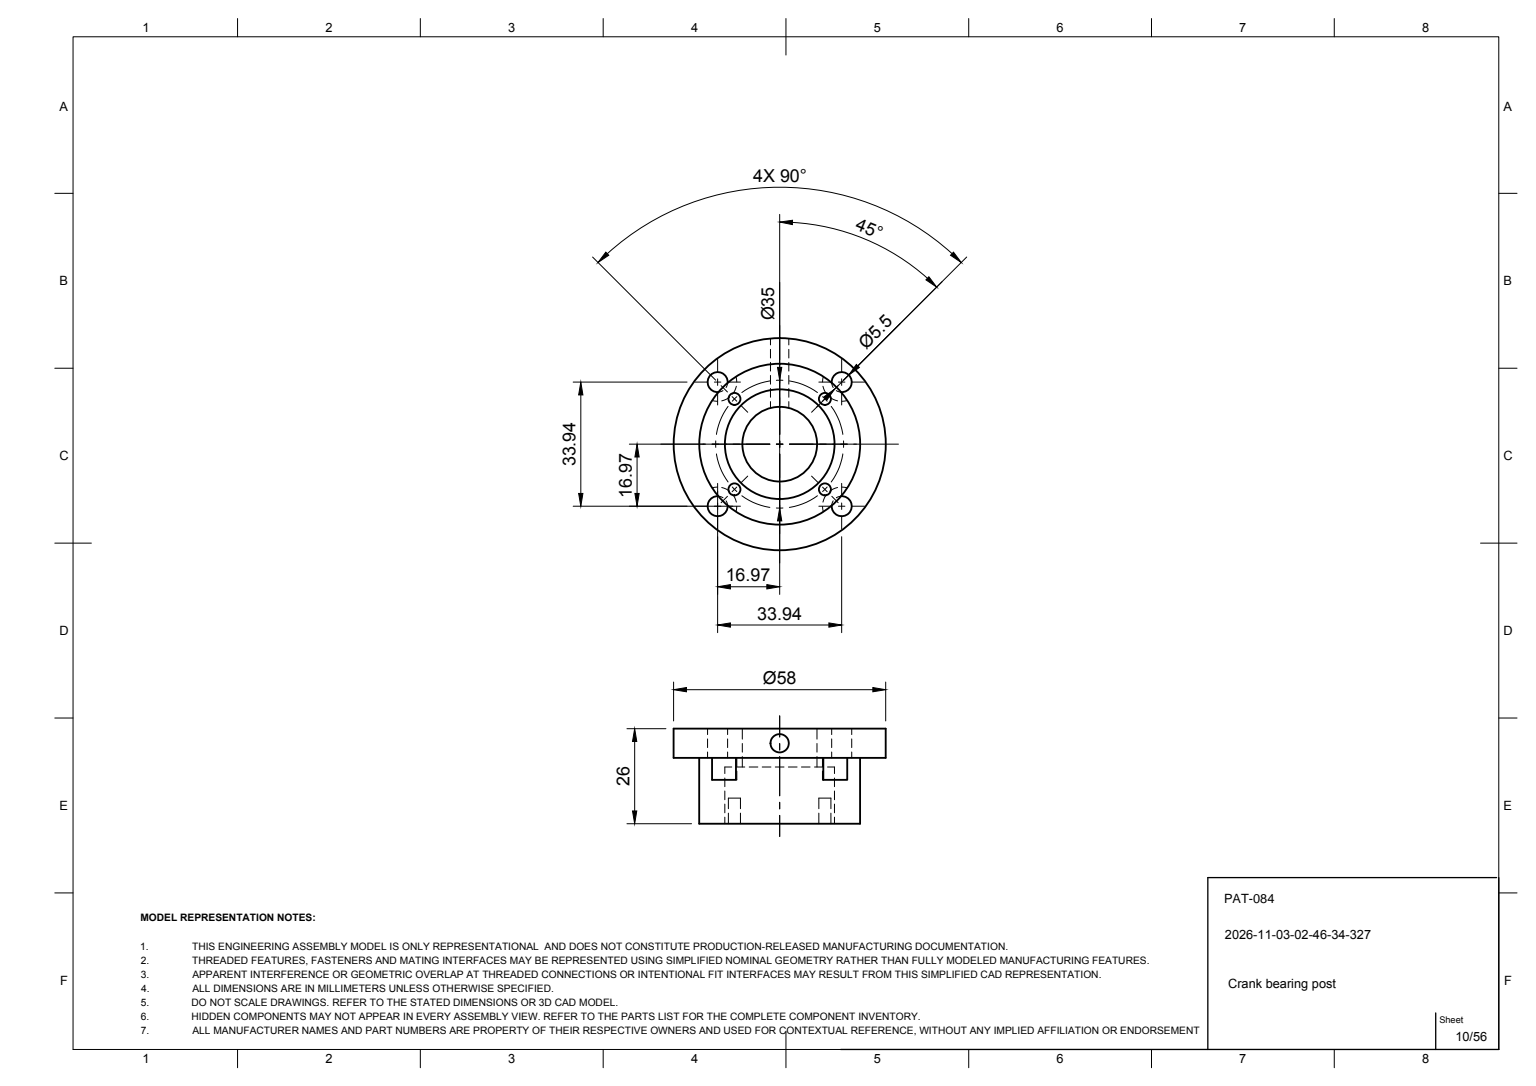
ISO-10303-21;
HEADER;
/* Generated by software containing ST-Developer
 * from STEP Tools, Inc. (www.steptools.com) 
 */

FILE_DESCRIPTION(
/* description */ ('Quick-return (Whitworth) mechanism'),
/* implementation_level */ '2;1');

FILE_NAME(
/* name */ 'Crank bearing post.step',
/* time_stamp */ '2026-10-28T03:25:57-07:00',
/* author */ (''),
/* organization */ (''),
/* preprocessor_version */ 'ST-DEVELOPER v20.2',
/* originating_system */ 'Autodesk Translation Framework v15.17.0.0',
/* authorisation */ '');

FILE_SCHEMA (('AUTOMOTIVE_DESIGN { 1 0 10303 214 3 1 1 }'));
ENDSEC;

DATA;
#10=MECHANICAL_DESIGN_GEOMETRIC_PRESENTATION_REPRESENTATION('',(#495),#14878);
#370=B_SPLINE_CURVE_WITH_KNOTS('',3,(#12386,#12387,#12388,#12389,#12390,
#12391,#12392,#12393,#12394,#12395),.UNSPECIFIED.,.F.,.F.,(4,2,2,2,4),(0.,
0.094594182476448,0.189188364952896,0.283770357603024,0.378352350253152),
 .UNSPECIFIED.);
#371=B_SPLINE_CURVE_WITH_KNOTS('',3,(#12396,#12397,#12398,#12399,#12400,
#12401,#12402,#12403,#12404,#12405,#12406,#12407,#12408,#12409,#12410,#12411,
#12412,#12413,#12414,#12415,#12416,#12417,#12418,#12419,#12420,#12421),
 .UNSPECIFIED.,.F.,.F.,(4,2,2,2,2,2,2,2,2,2,2,2,4),(0.378352350253152,0.472934342903279,
0.567516335553407,0.662110518029855,0.756704700506303,0.851298882982751,
0.945893065459199,1.04047505810933,1.13505705075945,1.22963904340958,1.32422103605971,
1.41881521853616,1.51340940101261),.UNSPECIFIED.);
#372=B_SPLINE_CURVE_WITH_KNOTS('',3,(#12425,#12426,#12427,#12428,#12429,
#12430,#12431,#12432,#12433,#12434,#12435,#12436,#12437,#12438,#12439,#12440,
#12441,#12442,#12443,#12444,#12445,#12446,#12447,#12448,#12449,#12450),
 .UNSPECIFIED.,.F.,.F.,(4,2,2,2,2,2,2,2,2,2,2,2,4),(0.,0.094221953570005,
0.18844390714001,0.282665684012033,0.376887460884057,0.47110923775608,0.565331014628104,
0.659552968198109,0.753774921768114,0.847996875338119,0.942218828908123,
1.03644060578015,1.13066238265217),.UNSPECIFIED.);
#373=B_SPLINE_CURVE_WITH_KNOTS('',3,(#12451,#12452,#12453,#12454,#12455,
#12456,#12457,#12458,#12459,#12460),.UNSPECIFIED.,.F.,.F.,(4,2,2,2,4),(1.13066238265217,
1.22488415952419,1.31910593639622,1.41332788996622,1.50754984353623),
 .UNSPECIFIED.);
#407=SHAPE_REPRESENTATION_RELATIONSHIP('SRR','None',#15075,#451);
#451=ADVANCED_BREP_SHAPE_REPRESENTATION('',(#547),#14832);
#495=STYLED_ITEM('',(#15406),#547);
#547=MANIFOLD_SOLID_BREP('Body1',#7849);
#648=FACE_BOUND('',#1665,.T.);
#649=FACE_BOUND('',#1666,.T.);
#650=FACE_BOUND('',#1667,.T.);
#651=FACE_BOUND('',#1668,.T.);
#652=FACE_BOUND('',#1669,.T.);
#653=FACE_BOUND('',#1677,.T.);
#654=FACE_BOUND('',#1679,.T.);
#655=FACE_BOUND('',#1681,.T.);
#656=FACE_BOUND('',#1683,.T.);
#657=FACE_BOUND('',#1684,.T.);
#658=FACE_BOUND('',#1685,.T.);
#659=FACE_BOUND('',#1686,.T.);
#660=FACE_BOUND('',#1687,.T.);
#661=FACE_BOUND('',#1689,.T.);
#662=FACE_BOUND('',#1690,.T.);
#663=FACE_BOUND('',#1691,.T.);
#664=FACE_BOUND('',#1692,.T.);
#665=FACE_BOUND('',#1693,.T.);
#819=PLANE('',#8559);
#820=PLANE('',#8563);
#821=PLANE('',#8567);
#822=PLANE('',#8571);
#823=PLANE('',#8575);
#824=PLANE('',#8580);
#825=PLANE('',#8585);
#826=PLANE('',#8590);
#827=PLANE('',#8592);
#828=PLANE('',#8616);
#829=PLANE('',#8622);
#830=PLANE('',#8623);
#1124=FACE_OUTER_BOUND('',#1647,.T.);
#1125=FACE_OUTER_BOUND('',#1648,.T.);
#1126=FACE_OUTER_BOUND('',#1649,.T.);
#1127=FACE_OUTER_BOUND('',#1650,.T.);
#1128=FACE_OUTER_BOUND('',#1651,.T.);
#1129=FACE_OUTER_BOUND('',#1652,.T.);
#1130=FACE_OUTER_BOUND('',#1653,.T.);
#1131=FACE_OUTER_BOUND('',#1654,.T.);
#1132=FACE_OUTER_BOUND('',#1655,.T.);
#1133=FACE_OUTER_BOUND('',#1656,.T.);
#1134=FACE_OUTER_BOUND('',#1657,.T.);
#1135=FACE_OUTER_BOUND('',#1658,.T.);
#1136=FACE_OUTER_BOUND('',#1659,.T.);
#1137=FACE_OUTER_BOUND('',#1660,.T.);
#1138=FACE_OUTER_BOUND('',#1661,.T.);
#1139=FACE_OUTER_BOUND('',#1662,.T.);
#1140=FACE_OUTER_BOUND('',#1663,.T.);
#1141=FACE_OUTER_BOUND('',#1664,.T.);
#1142=FACE_OUTER_BOUND('',#1670,.T.);
#1143=FACE_OUTER_BOUND('',#1671,.T.);
#1144=FACE_OUTER_BOUND('',#1672,.T.);
#1145=FACE_OUTER_BOUND('',#1673,.T.);
#1146=FACE_OUTER_BOUND('',#1674,.T.);
#1147=FACE_OUTER_BOUND('',#1675,.T.);
#1148=FACE_OUTER_BOUND('',#1676,.T.);
#1149=FACE_OUTER_BOUND('',#1678,.T.);
#1150=FACE_OUTER_BOUND('',#1680,.T.);
#1151=FACE_OUTER_BOUND('',#1682,.T.);
#1152=FACE_OUTER_BOUND('',#1688,.T.);
#1647=EDGE_LOOP('',(#5602,#5603,#5604,#5605,#5606,#5607));
#1648=EDGE_LOOP('',(#5608,#5609,#5610,#5611));
#1649=EDGE_LOOP('',(#5612));
#1650=EDGE_LOOP('',(#5613,#5614,#5615,#5616));
#1651=EDGE_LOOP('',(#5617));
#1652=EDGE_LOOP('',(#5618,#5619,#5620,#5621));
#1653=EDGE_LOOP('',(#5622));
#1654=EDGE_LOOP('',(#5623,#5624,#5625,#5626));
#1655=EDGE_LOOP('',(#5627));
#1656=EDGE_LOOP('',(#5628,#5629,#5630,#5631));
#1657=EDGE_LOOP('',(#5632,#5633));
#1658=EDGE_LOOP('',(#5634,#5635,#5636,#5637));
#1659=EDGE_LOOP('',(#5638,#5639));
#1660=EDGE_LOOP('',(#5640,#5641,#5642,#5643));
#1661=EDGE_LOOP('',(#5644,#5645));
#1662=EDGE_LOOP('',(#5646,#5647,#5648,#5649));
#1663=EDGE_LOOP('',(#5650,#5651));
#1664=EDGE_LOOP('',(#5652));
#1665=EDGE_LOOP('',(#5653,#5654,#5655,#5656,#5657,#5658,#5659,#5660,#5661));
#1666=EDGE_LOOP('',(#5662));
#1667=EDGE_LOOP('',(#5663));
#1668=EDGE_LOOP('',(#5664));
#1669=EDGE_LOOP('',(#5665));
#1670=EDGE_LOOP('',(#5666,#5667,#5668,#5669));
#1671=EDGE_LOOP('',(#5670,#5671,#5672,#5673));
#1672=EDGE_LOOP('',(#5674,#5675,#5676,#5677));
#1673=EDGE_LOOP('',(#5678,#5679,#5680,#5681));
#1674=EDGE_LOOP('',(#5682,#5683,#5684,#5685,#5686,#5687,#5688,#5689,#5690,
#5691,#5692,#5693,#5694,#5695,#5696,#5697,#5698,#5699,#5700,#5701));
#1675=EDGE_LOOP('',(#5702,#5703,#5704,#5705));
#1676=EDGE_LOOP('',(#5706));
#1677=EDGE_LOOP('',(#5707));
#1678=EDGE_LOOP('',(#5708,#5709,#5710,#5711));
#1679=EDGE_LOOP('',(#5712,#5713));
#1680=EDGE_LOOP('',(#5714,#5715,#5716,#5717));
#1681=EDGE_LOOP('',(#5718,#5719));
#1682=EDGE_LOOP('',(#5720));
#1683=EDGE_LOOP('',(#5721));
#1684=EDGE_LOOP('',(#5722));
#1685=EDGE_LOOP('',(#5723));
#1686=EDGE_LOOP('',(#5724));
#1687=EDGE_LOOP('',(#5725));
#1688=EDGE_LOOP('',(#5726));
#1689=EDGE_LOOP('',(#5727));
#1690=EDGE_LOOP('',(#5728));
#1691=EDGE_LOOP('',(#5729));
#1692=EDGE_LOOP('',(#5730));
#1693=EDGE_LOOP('',(#5731));
#2250=LINE('',#12423,#2773);
#2251=LINE('',#12465,#2774);
#2252=LINE('',#12472,#2775);
#2253=LINE('',#12479,#2776);
#2254=LINE('',#12486,#2777);
#2255=LINE('',#12492,#2778);
#2256=LINE('',#12496,#2779);
#2257=LINE('',#12503,#2780);
#2258=LINE('',#12507,#2781);
#2259=LINE('',#12514,#2782);
#2260=LINE('',#12518,#2783);
#2261=LINE('',#12525,#2784);
#2262=LINE('',#12529,#2785);
#2263=LINE('',#12553,#2786);
#2264=LINE('',#12557,#2787);
#2265=LINE('',#12561,#2788);
#2266=LINE('',#12565,#2789);
#2267=LINE('',#12569,#2790);
#2268=LINE('',#12574,#2791);
#2269=LINE('',#12581,#2792);
#2270=LINE('',#12585,#2793);
#2773=VECTOR('',#9821,0.25);
#2774=VECTOR('',#9826,0.165);
#2775=VECTOR('',#9835,0.165);
#2776=VECTOR('',#9844,0.165);
#2777=VECTOR('',#9853,0.165);
#2778=VECTOR('',#9860,1.);
#2779=VECTOR('',#9863,1.);
#2780=VECTOR('',#9872,1.);
#2781=VECTOR('',#9875,1.);
#2782=VECTOR('',#9884,1.);
#2783=VECTOR('',#9887,1.);
#2784=VECTOR('',#9896,1.);
#2785=VECTOR('',#9899,1.);
#2786=VECTOR('',#9932,0.275);
#2787=VECTOR('',#9937,0.275);
#2788=VECTOR('',#9942,0.275);
#2789=VECTOR('',#9947,0.275);
#2790=VECTOR('',#9952,2.2);
#2791=VECTOR('',#9957,1.5);
#2792=VECTOR('',#9966,2.9);
#2793=VECTOR('',#9971,1.02);
#3302=CIRCLE('',#8557,0.165);
#3303=CIRCLE('',#8558,0.165);
#3304=CIRCLE('',#8561,0.165);
#3305=CIRCLE('',#8562,0.165);
#3306=CIRCLE('',#8565,0.165);
#3307=CIRCLE('',#8566,0.165);
#3308=CIRCLE('',#8569,0.165);
#3309=CIRCLE('',#8570,0.165);
#3310=CIRCLE('',#8573,0.525);
#3311=CIRCLE('',#8574,0.525);
#3312=CIRCLE('',#8576,2.2);
#3313=CIRCLE('',#8578,0.525);
#3314=CIRCLE('',#8579,0.525);
#3315=CIRCLE('',#8581,2.2);
#3316=CIRCLE('',#8583,0.525);
#3317=CIRCLE('',#8584,0.525);
#3318=CIRCLE('',#8586,2.2);
#3319=CIRCLE('',#8588,0.525);
#3320=CIRCLE('',#8589,0.525);
#3321=CIRCLE('',#8591,2.2);
#3322=CIRCLE('',#8593,2.9);
#3323=CIRCLE('',#8594,2.2);
#3324=CIRCLE('',#8595,2.2);
#3325=CIRCLE('',#8596,2.2);
#3326=CIRCLE('',#8597,2.2);
#3327=CIRCLE('',#8598,2.2);
#3328=CIRCLE('',#8599,0.275);
#3329=CIRCLE('',#8600,0.275);
#3330=CIRCLE('',#8601,0.275);
#3331=CIRCLE('',#8602,0.275);
#3332=CIRCLE('',#8604,0.275);
#3333=CIRCLE('',#8606,0.275);
#3334=CIRCLE('',#8608,0.275);
#3335=CIRCLE('',#8610,0.275);
#3336=CIRCLE('',#8612,2.2);
#3337=CIRCLE('',#8614,1.5);
#3338=CIRCLE('',#8615,1.5);
#3339=CIRCLE('',#8617,1.02);
#3340=CIRCLE('',#8619,2.9);
#3341=CIRCLE('',#8621,1.02);
#3745=VERTEX_POINT('',#12384);
#3746=VERTEX_POINT('',#12385);
#3747=VERTEX_POINT('',#12422);
#3748=VERTEX_POINT('',#12424);
#3749=VERTEX_POINT('',#12462);
#3750=VERTEX_POINT('',#12464);
#3751=VERTEX_POINT('',#12469);
#3752=VERTEX_POINT('',#12471);
#3753=VERTEX_POINT('',#12476);
#3754=VERTEX_POINT('',#12478);
#3755=VERTEX_POINT('',#12483);
#3756=VERTEX_POINT('',#12485);
#3757=VERTEX_POINT('',#12490);
#3758=VERTEX_POINT('',#12491);
#3759=VERTEX_POINT('',#12493);
#3760=VERTEX_POINT('',#12495);
#3761=VERTEX_POINT('',#12501);
#3762=VERTEX_POINT('',#12502);
#3763=VERTEX_POINT('',#12504);
#3764=VERTEX_POINT('',#12506);
#3765=VERTEX_POINT('',#12512);
#3766=VERTEX_POINT('',#12513);
#3767=VERTEX_POINT('',#12515);
#3768=VERTEX_POINT('',#12517);
#3769=VERTEX_POINT('',#12523);
#3770=VERTEX_POINT('',#12524);
#3771=VERTEX_POINT('',#12526);
#3772=VERTEX_POINT('',#12528);
#3773=VERTEX_POINT('',#12534);
#3774=VERTEX_POINT('',#12536);
#3775=VERTEX_POINT('',#12542);
#3776=VERTEX_POINT('',#12544);
#3777=VERTEX_POINT('',#12546);
#3778=VERTEX_POINT('',#12548);
#3779=VERTEX_POINT('',#12551);
#3780=VERTEX_POINT('',#12555);
#3781=VERTEX_POINT('',#12559);
#3782=VERTEX_POINT('',#12563);
#3783=VERTEX_POINT('',#12567);
#3784=VERTEX_POINT('',#12571);
#3785=VERTEX_POINT('',#12573);
#3786=VERTEX_POINT('',#12577);
#3787=VERTEX_POINT('',#12580);
#3788=VERTEX_POINT('',#12584);
#4458=EDGE_CURVE('',#3745,#3746,#370,.T.);
#4459=EDGE_CURVE('',#3746,#3745,#371,.T.);
#4460=EDGE_CURVE('',#3746,#3747,#2250,.T.);
#4461=EDGE_CURVE('',#3748,#3747,#372,.T.);
#4462=EDGE_CURVE('',#3747,#3748,#373,.T.);
#4463=EDGE_CURVE('',#3749,#3749,#3302,.T.);
#4464=EDGE_CURVE('',#3749,#3750,#2251,.T.);
#4465=EDGE_CURVE('',#3750,#3750,#3303,.T.);
#4466=EDGE_CURVE('',#3751,#3751,#3304,.T.);
#4467=EDGE_CURVE('',#3751,#3752,#2252,.T.);
#4468=EDGE_CURVE('',#3752,#3752,#3305,.T.);
#4469=EDGE_CURVE('',#3753,#3753,#3306,.T.);
#4470=EDGE_CURVE('',#3753,#3754,#2253,.T.);
#4471=EDGE_CURVE('',#3754,#3754,#3307,.T.);
#4472=EDGE_CURVE('',#3755,#3755,#3308,.T.);
#4473=EDGE_CURVE('',#3755,#3756,#2254,.T.);
#4474=EDGE_CURVE('',#3756,#3756,#3309,.T.);
#4475=EDGE_CURVE('',#3757,#3758,#2255,.T.);
#4476=EDGE_CURVE('',#3757,#3759,#3310,.T.);
#4477=EDGE_CURVE('',#3760,#3759,#2256,.T.);
#4478=EDGE_CURVE('',#3758,#3760,#3311,.T.);
#4479=EDGE_CURVE('',#3759,#3757,#3312,.T.);
#4480=EDGE_CURVE('',#3761,#3762,#2257,.T.);
#4481=EDGE_CURVE('',#3761,#3763,#3313,.T.);
#4482=EDGE_CURVE('',#3764,#3763,#2258,.T.);
#4483=EDGE_CURVE('',#3762,#3764,#3314,.T.);
#4484=EDGE_CURVE('',#3763,#3761,#3315,.T.);
#4485=EDGE_CURVE('',#3765,#3766,#2259,.T.);
#4486=EDGE_CURVE('',#3765,#3767,#3316,.T.);
#4487=EDGE_CURVE('',#3768,#3767,#2260,.T.);
#4488=EDGE_CURVE('',#3766,#3768,#3317,.T.);
#4489=EDGE_CURVE('',#3767,#3765,#3318,.T.);
#4490=EDGE_CURVE('',#3769,#3770,#2261,.T.);
#4491=EDGE_CURVE('',#3769,#3771,#3319,.T.);
#4492=EDGE_CURVE('',#3772,#3771,#2262,.T.);
#4493=EDGE_CURVE('',#3770,#3772,#3320,.T.);
#4494=EDGE_CURVE('',#3771,#3769,#3321,.T.);
#4495=EDGE_CURVE('',#3773,#3773,#3322,.T.);
#4496=EDGE_CURVE('',#3762,#3774,#3323,.T.);
#4497=EDGE_CURVE('',#3766,#3764,#3324,.T.);
#4498=EDGE_CURVE('',#3770,#3768,#3325,.T.);
#4499=EDGE_CURVE('',#3758,#3772,#3326,.T.);
#4500=EDGE_CURVE('',#3774,#3760,#3327,.T.);
#4501=EDGE_CURVE('',#3775,#3775,#3328,.T.);
#4502=EDGE_CURVE('',#3776,#3776,#3329,.T.);
#4503=EDGE_CURVE('',#3777,#3777,#3330,.T.);
#4504=EDGE_CURVE('',#3778,#3778,#3331,.T.);
#4505=EDGE_CURVE('',#3779,#3779,#3332,.T.);
#4506=EDGE_CURVE('',#3779,#3775,#2263,.T.);
#4507=EDGE_CURVE('',#3780,#3780,#3333,.T.);
#4508=EDGE_CURVE('',#3780,#3776,#2264,.T.);
#4509=EDGE_CURVE('',#3781,#3781,#3334,.T.);
#4510=EDGE_CURVE('',#3781,#3777,#2265,.T.);
#4511=EDGE_CURVE('',#3782,#3782,#3335,.T.);
#4512=EDGE_CURVE('',#3782,#3778,#2266,.T.);
#4513=EDGE_CURVE('',#3783,#3783,#3336,.T.);
#4514=EDGE_CURVE('',#3783,#3774,#2267,.T.);
#4515=EDGE_CURVE('',#3784,#3784,#3337,.T.);
#4516=EDGE_CURVE('',#3784,#3785,#2268,.T.);
#4517=EDGE_CURVE('',#3785,#3785,#3338,.T.);
#4518=EDGE_CURVE('',#3786,#3786,#3339,.T.);
#4519=EDGE_CURVE('',#3773,#3787,#2269,.T.);
#4520=EDGE_CURVE('',#3787,#3787,#3340,.T.);
#4521=EDGE_CURVE('',#3786,#3788,#2270,.T.);
#4522=EDGE_CURVE('',#3788,#3788,#3341,.T.);
#5602=ORIENTED_EDGE('',*,*,#4458,.F.);
#5603=ORIENTED_EDGE('',*,*,#4459,.F.);
#5604=ORIENTED_EDGE('',*,*,#4460,.T.);
#5605=ORIENTED_EDGE('',*,*,#4461,.F.);
#5606=ORIENTED_EDGE('',*,*,#4462,.F.);
#5607=ORIENTED_EDGE('',*,*,#4460,.F.);
#5608=ORIENTED_EDGE('',*,*,#4463,.F.);
#5609=ORIENTED_EDGE('',*,*,#4464,.T.);
#5610=ORIENTED_EDGE('',*,*,#4465,.F.);
#5611=ORIENTED_EDGE('',*,*,#4464,.F.);
#5612=ORIENTED_EDGE('',*,*,#4463,.T.);
#5613=ORIENTED_EDGE('',*,*,#4466,.F.);
#5614=ORIENTED_EDGE('',*,*,#4467,.T.);
#5615=ORIENTED_EDGE('',*,*,#4468,.F.);
#5616=ORIENTED_EDGE('',*,*,#4467,.F.);
#5617=ORIENTED_EDGE('',*,*,#4466,.T.);
#5618=ORIENTED_EDGE('',*,*,#4469,.F.);
#5619=ORIENTED_EDGE('',*,*,#4470,.T.);
#5620=ORIENTED_EDGE('',*,*,#4471,.F.);
#5621=ORIENTED_EDGE('',*,*,#4470,.F.);
#5622=ORIENTED_EDGE('',*,*,#4469,.T.);
#5623=ORIENTED_EDGE('',*,*,#4472,.F.);
#5624=ORIENTED_EDGE('',*,*,#4473,.T.);
#5625=ORIENTED_EDGE('',*,*,#4474,.F.);
#5626=ORIENTED_EDGE('',*,*,#4473,.F.);
#5627=ORIENTED_EDGE('',*,*,#4472,.T.);
#5628=ORIENTED_EDGE('',*,*,#4475,.F.);
#5629=ORIENTED_EDGE('',*,*,#4476,.T.);
#5630=ORIENTED_EDGE('',*,*,#4477,.F.);
#5631=ORIENTED_EDGE('',*,*,#4478,.F.);
#5632=ORIENTED_EDGE('',*,*,#4479,.F.);
#5633=ORIENTED_EDGE('',*,*,#4476,.F.);
#5634=ORIENTED_EDGE('',*,*,#4480,.F.);
#5635=ORIENTED_EDGE('',*,*,#4481,.T.);
#5636=ORIENTED_EDGE('',*,*,#4482,.F.);
#5637=ORIENTED_EDGE('',*,*,#4483,.F.);
#5638=ORIENTED_EDGE('',*,*,#4484,.F.);
#5639=ORIENTED_EDGE('',*,*,#4481,.F.);
#5640=ORIENTED_EDGE('',*,*,#4485,.F.);
#5641=ORIENTED_EDGE('',*,*,#4486,.T.);
#5642=ORIENTED_EDGE('',*,*,#4487,.F.);
#5643=ORIENTED_EDGE('',*,*,#4488,.F.);
#5644=ORIENTED_EDGE('',*,*,#4489,.F.);
#5645=ORIENTED_EDGE('',*,*,#4486,.F.);
#5646=ORIENTED_EDGE('',*,*,#4490,.F.);
#5647=ORIENTED_EDGE('',*,*,#4491,.T.);
#5648=ORIENTED_EDGE('',*,*,#4492,.F.);
#5649=ORIENTED_EDGE('',*,*,#4493,.F.);
#5650=ORIENTED_EDGE('',*,*,#4494,.F.);
#5651=ORIENTED_EDGE('',*,*,#4491,.F.);
#5652=ORIENTED_EDGE('',*,*,#4495,.T.);
#5653=ORIENTED_EDGE('',*,*,#4496,.F.);
#5654=ORIENTED_EDGE('',*,*,#4483,.T.);
#5655=ORIENTED_EDGE('',*,*,#4497,.F.);
#5656=ORIENTED_EDGE('',*,*,#4488,.T.);
#5657=ORIENTED_EDGE('',*,*,#4498,.F.);
#5658=ORIENTED_EDGE('',*,*,#4493,.T.);
#5659=ORIENTED_EDGE('',*,*,#4499,.F.);
#5660=ORIENTED_EDGE('',*,*,#4478,.T.);
#5661=ORIENTED_EDGE('',*,*,#4500,.F.);
#5662=ORIENTED_EDGE('',*,*,#4501,.T.);
#5663=ORIENTED_EDGE('',*,*,#4502,.T.);
#5664=ORIENTED_EDGE('',*,*,#4503,.T.);
#5665=ORIENTED_EDGE('',*,*,#4504,.T.);
#5666=ORIENTED_EDGE('',*,*,#4505,.F.);
#5667=ORIENTED_EDGE('',*,*,#4506,.T.);
#5668=ORIENTED_EDGE('',*,*,#4501,.F.);
#5669=ORIENTED_EDGE('',*,*,#4506,.F.);
#5670=ORIENTED_EDGE('',*,*,#4507,.F.);
#5671=ORIENTED_EDGE('',*,*,#4508,.T.);
#5672=ORIENTED_EDGE('',*,*,#4502,.F.);
#5673=ORIENTED_EDGE('',*,*,#4508,.F.);
#5674=ORIENTED_EDGE('',*,*,#4509,.F.);
#5675=ORIENTED_EDGE('',*,*,#4510,.T.);
#5676=ORIENTED_EDGE('',*,*,#4503,.F.);
#5677=ORIENTED_EDGE('',*,*,#4510,.F.);
#5678=ORIENTED_EDGE('',*,*,#4511,.F.);
#5679=ORIENTED_EDGE('',*,*,#4512,.T.);
#5680=ORIENTED_EDGE('',*,*,#4504,.F.);
#5681=ORIENTED_EDGE('',*,*,#4512,.F.);
#5682=ORIENTED_EDGE('',*,*,#4513,.F.);
#5683=ORIENTED_EDGE('',*,*,#4514,.T.);
#5684=ORIENTED_EDGE('',*,*,#4500,.T.);
#5685=ORIENTED_EDGE('',*,*,#4477,.T.);
#5686=ORIENTED_EDGE('',*,*,#4479,.T.);
#5687=ORIENTED_EDGE('',*,*,#4475,.T.);
#5688=ORIENTED_EDGE('',*,*,#4499,.T.);
#5689=ORIENTED_EDGE('',*,*,#4492,.T.);
#5690=ORIENTED_EDGE('',*,*,#4494,.T.);
#5691=ORIENTED_EDGE('',*,*,#4490,.T.);
#5692=ORIENTED_EDGE('',*,*,#4498,.T.);
#5693=ORIENTED_EDGE('',*,*,#4487,.T.);
#5694=ORIENTED_EDGE('',*,*,#4489,.T.);
#5695=ORIENTED_EDGE('',*,*,#4485,.T.);
#5696=ORIENTED_EDGE('',*,*,#4497,.T.);
#5697=ORIENTED_EDGE('',*,*,#4482,.T.);
#5698=ORIENTED_EDGE('',*,*,#4484,.T.);
#5699=ORIENTED_EDGE('',*,*,#4480,.T.);
#5700=ORIENTED_EDGE('',*,*,#4496,.T.);
#5701=ORIENTED_EDGE('',*,*,#4514,.F.);
#5702=ORIENTED_EDGE('',*,*,#4515,.F.);
#5703=ORIENTED_EDGE('',*,*,#4516,.T.);
#5704=ORIENTED_EDGE('',*,*,#4517,.F.);
#5705=ORIENTED_EDGE('',*,*,#4516,.F.);
#5706=ORIENTED_EDGE('',*,*,#4515,.T.);
#5707=ORIENTED_EDGE('',*,*,#4518,.F.);
#5708=ORIENTED_EDGE('',*,*,#4495,.F.);
#5709=ORIENTED_EDGE('',*,*,#4519,.T.);
#5710=ORIENTED_EDGE('',*,*,#4520,.T.);
#5711=ORIENTED_EDGE('',*,*,#4519,.F.);
#5712=ORIENTED_EDGE('',*,*,#4461,.T.);
#5713=ORIENTED_EDGE('',*,*,#4462,.T.);
#5714=ORIENTED_EDGE('',*,*,#4518,.T.);
#5715=ORIENTED_EDGE('',*,*,#4521,.T.);
#5716=ORIENTED_EDGE('',*,*,#4522,.T.);
#5717=ORIENTED_EDGE('',*,*,#4521,.F.);
#5718=ORIENTED_EDGE('',*,*,#4458,.T.);
#5719=ORIENTED_EDGE('',*,*,#4459,.T.);
#5720=ORIENTED_EDGE('',*,*,#4513,.T.);
#5721=ORIENTED_EDGE('',*,*,#4517,.T.);
#5722=ORIENTED_EDGE('',*,*,#4474,.T.);
#5723=ORIENTED_EDGE('',*,*,#4471,.T.);
#5724=ORIENTED_EDGE('',*,*,#4468,.T.);
#5725=ORIENTED_EDGE('',*,*,#4465,.T.);
#5726=ORIENTED_EDGE('',*,*,#4520,.F.);
#5727=ORIENTED_EDGE('',*,*,#4522,.F.);
#5728=ORIENTED_EDGE('',*,*,#4511,.T.);
#5729=ORIENTED_EDGE('',*,*,#4509,.T.);
#5730=ORIENTED_EDGE('',*,*,#4507,.T.);
#5731=ORIENTED_EDGE('',*,*,#4505,.T.);
#7250=CYLINDRICAL_SURFACE('',#8555,0.25);
#7251=CYLINDRICAL_SURFACE('',#8556,0.165);
#7252=CYLINDRICAL_SURFACE('',#8560,0.165);
#7253=CYLINDRICAL_SURFACE('',#8564,0.165);
#7254=CYLINDRICAL_SURFACE('',#8568,0.165);
#7255=CYLINDRICAL_SURFACE('',#8572,0.525);
#7256=CYLINDRICAL_SURFACE('',#8577,0.525);
#7257=CYLINDRICAL_SURFACE('',#8582,0.525);
#7258=CYLINDRICAL_SURFACE('',#8587,0.525);
#7259=CYLINDRICAL_SURFACE('',#8603,0.275);
#7260=CYLINDRICAL_SURFACE('',#8605,0.275);
#7261=CYLINDRICAL_SURFACE('',#8607,0.275);
#7262=CYLINDRICAL_SURFACE('',#8609,0.275);
#7263=CYLINDRICAL_SURFACE('',#8611,2.2);
#7264=CYLINDRICAL_SURFACE('',#8613,1.5);
#7265=CYLINDRICAL_SURFACE('',#8618,2.9);
#7266=CYLINDRICAL_SURFACE('',#8620,1.02);
#7455=ADVANCED_FACE('',(#1124),#7250,.F.);
#7456=ADVANCED_FACE('',(#1125),#7251,.F.);
#7457=ADVANCED_FACE('',(#1126),#819,.T.);
#7458=ADVANCED_FACE('',(#1127),#7252,.F.);
#7459=ADVANCED_FACE('',(#1128),#820,.T.);
#7460=ADVANCED_FACE('',(#1129),#7253,.F.);
#7461=ADVANCED_FACE('',(#1130),#821,.T.);
#7462=ADVANCED_FACE('',(#1131),#7254,.F.);
#7463=ADVANCED_FACE('',(#1132),#822,.T.);
#7464=ADVANCED_FACE('',(#1133),#7255,.F.);
#7465=ADVANCED_FACE('',(#1134),#823,.F.);
#7466=ADVANCED_FACE('',(#1135),#7256,.F.);
#7467=ADVANCED_FACE('',(#1136),#824,.F.);
#7468=ADVANCED_FACE('',(#1137),#7257,.F.);
#7469=ADVANCED_FACE('',(#1138),#825,.F.);
#7470=ADVANCED_FACE('',(#1139),#7258,.F.);
#7471=ADVANCED_FACE('',(#1140),#826,.F.);
#7472=ADVANCED_FACE('',(#1141,#648,#649,#650,#651,#652),#827,.T.);
#7473=ADVANCED_FACE('',(#1142),#7259,.F.);
#7474=ADVANCED_FACE('',(#1143),#7260,.F.);
#7475=ADVANCED_FACE('',(#1144),#7261,.F.);
#7476=ADVANCED_FACE('',(#1145),#7262,.F.);
#7477=ADVANCED_FACE('',(#1146),#7263,.T.);
#7478=ADVANCED_FACE('',(#1147),#7264,.F.);
#7479=ADVANCED_FACE('',(#1148,#653),#828,.T.);
#7480=ADVANCED_FACE('',(#1149,#654),#7265,.T.);
#7481=ADVANCED_FACE('',(#1150,#655),#7266,.F.);
#7482=ADVANCED_FACE('',(#1151,#656,#657,#658,#659,#660),#829,.T.);
#7483=ADVANCED_FACE('',(#1152,#661,#662,#663,#664,#665),#830,.F.);
#7849=CLOSED_SHELL('',(#7455,#7456,#7457,#7458,#7459,#7460,#7461,#7462,
#7463,#7464,#7465,#7466,#7467,#7468,#7469,#7470,#7471,#7472,#7473,#7474,
#7475,#7476,#7477,#7478,#7479,#7480,#7481,#7482,#7483));
#8554=AXIS2_PLACEMENT_3D('',#12382,#9817,#9818);
#8555=AXIS2_PLACEMENT_3D('',#12383,#9819,#9820);
#8556=AXIS2_PLACEMENT_3D('',#12461,#9822,#9823);
#8557=AXIS2_PLACEMENT_3D('',#12463,#9824,#9825);
#8558=AXIS2_PLACEMENT_3D('',#12466,#9827,#9828);
#8559=AXIS2_PLACEMENT_3D('',#12467,#9829,#9830);
#8560=AXIS2_PLACEMENT_3D('',#12468,#9831,#9832);
#8561=AXIS2_PLACEMENT_3D('',#12470,#9833,#9834);
#8562=AXIS2_PLACEMENT_3D('',#12473,#9836,#9837);
#8563=AXIS2_PLACEMENT_3D('',#12474,#9838,#9839);
#8564=AXIS2_PLACEMENT_3D('',#12475,#9840,#9841);
#8565=AXIS2_PLACEMENT_3D('',#12477,#9842,#9843);
#8566=AXIS2_PLACEMENT_3D('',#12480,#9845,#9846);
#8567=AXIS2_PLACEMENT_3D('',#12481,#9847,#9848);
#8568=AXIS2_PLACEMENT_3D('',#12482,#9849,#9850);
#8569=AXIS2_PLACEMENT_3D('',#12484,#9851,#9852);
#8570=AXIS2_PLACEMENT_3D('',#12487,#9854,#9855);
#8571=AXIS2_PLACEMENT_3D('',#12488,#9856,#9857);
#8572=AXIS2_PLACEMENT_3D('',#12489,#9858,#9859);
#8573=AXIS2_PLACEMENT_3D('',#12494,#9861,#9862);
#8574=AXIS2_PLACEMENT_3D('',#12497,#9864,#9865);
#8575=AXIS2_PLACEMENT_3D('',#12498,#9866,#9867);
#8576=AXIS2_PLACEMENT_3D('',#12499,#9868,#9869);
#8577=AXIS2_PLACEMENT_3D('',#12500,#9870,#9871);
#8578=AXIS2_PLACEMENT_3D('',#12505,#9873,#9874);
#8579=AXIS2_PLACEMENT_3D('',#12508,#9876,#9877);
#8580=AXIS2_PLACEMENT_3D('',#12509,#9878,#9879);
#8581=AXIS2_PLACEMENT_3D('',#12510,#9880,#9881);
#8582=AXIS2_PLACEMENT_3D('',#12511,#9882,#9883);
#8583=AXIS2_PLACEMENT_3D('',#12516,#9885,#9886);
#8584=AXIS2_PLACEMENT_3D('',#12519,#9888,#9889);
#8585=AXIS2_PLACEMENT_3D('',#12520,#9890,#9891);
#8586=AXIS2_PLACEMENT_3D('',#12521,#9892,#9893);
#8587=AXIS2_PLACEMENT_3D('',#12522,#9894,#9895);
#8588=AXIS2_PLACEMENT_3D('',#12527,#9897,#9898);
#8589=AXIS2_PLACEMENT_3D('',#12530,#9900,#9901);
#8590=AXIS2_PLACEMENT_3D('',#12531,#9902,#9903);
#8591=AXIS2_PLACEMENT_3D('',#12532,#9904,#9905);
#8592=AXIS2_PLACEMENT_3D('',#12533,#9906,#9907);
#8593=AXIS2_PLACEMENT_3D('',#12535,#9908,#9909);
#8594=AXIS2_PLACEMENT_3D('',#12537,#9910,#9911);
#8595=AXIS2_PLACEMENT_3D('',#12538,#9912,#9913);
#8596=AXIS2_PLACEMENT_3D('',#12539,#9914,#9915);
#8597=AXIS2_PLACEMENT_3D('',#12540,#9916,#9917);
#8598=AXIS2_PLACEMENT_3D('',#12541,#9918,#9919);
#8599=AXIS2_PLACEMENT_3D('',#12543,#9920,#9921);
#8600=AXIS2_PLACEMENT_3D('',#12545,#9922,#9923);
#8601=AXIS2_PLACEMENT_3D('',#12547,#9924,#9925);
#8602=AXIS2_PLACEMENT_3D('',#12549,#9926,#9927);
#8603=AXIS2_PLACEMENT_3D('',#12550,#9928,#9929);
#8604=AXIS2_PLACEMENT_3D('',#12552,#9930,#9931);
#8605=AXIS2_PLACEMENT_3D('',#12554,#9933,#9934);
#8606=AXIS2_PLACEMENT_3D('',#12556,#9935,#9936);
#8607=AXIS2_PLACEMENT_3D('',#12558,#9938,#9939);
#8608=AXIS2_PLACEMENT_3D('',#12560,#9940,#9941);
#8609=AXIS2_PLACEMENT_3D('',#12562,#9943,#9944);
#8610=AXIS2_PLACEMENT_3D('',#12564,#9945,#9946);
#8611=AXIS2_PLACEMENT_3D('',#12566,#9948,#9949);
#8612=AXIS2_PLACEMENT_3D('',#12568,#9950,#9951);
#8613=AXIS2_PLACEMENT_3D('',#12570,#9953,#9954);
#8614=AXIS2_PLACEMENT_3D('',#12572,#9955,#9956);
#8615=AXIS2_PLACEMENT_3D('',#12575,#9958,#9959);
#8616=AXIS2_PLACEMENT_3D('',#12576,#9960,#9961);
#8617=AXIS2_PLACEMENT_3D('',#12578,#9962,#9963);
#8618=AXIS2_PLACEMENT_3D('',#12579,#9964,#9965);
#8619=AXIS2_PLACEMENT_3D('',#12582,#9967,#9968);
#8620=AXIS2_PLACEMENT_3D('',#12583,#9969,#9970);
#8621=AXIS2_PLACEMENT_3D('',#12586,#9972,#9973);
#8622=AXIS2_PLACEMENT_3D('',#12587,#9974,#9975);
#8623=AXIS2_PLACEMENT_3D('',#12588,#9976,#9977);
#9817=DIRECTION('axis',(0.,0.,1.));
#9818=DIRECTION('refdir',(1.,0.,0.));
#9819=DIRECTION('center_axis',(1.,0.,0.));
#9820=DIRECTION('ref_axis',(0.,0.,-1.));
#9821=DIRECTION('',(1.,0.,0.));
#9822=DIRECTION('center_axis',(0.,0.,1.));
#9823=DIRECTION('ref_axis',(1.,0.,0.));
#9824=DIRECTION('center_axis',(0.,0.,1.));
#9825=DIRECTION('ref_axis',(1.,0.,0.));
#9826=DIRECTION('',(0.,0.,1.));
#9827=DIRECTION('center_axis',(0.,0.,-1.));
#9828=DIRECTION('ref_axis',(1.,0.,0.));
#9829=DIRECTION('center_axis',(0.,0.,1.));
#9830=DIRECTION('ref_axis',(1.,0.,0.));
#9831=DIRECTION('center_axis',(0.,0.,1.));
#9832=DIRECTION('ref_axis',(1.,0.,0.));
#9833=DIRECTION('center_axis',(0.,0.,1.));
#9834=DIRECTION('ref_axis',(1.,0.,0.));
#9835=DIRECTION('',(0.,0.,1.));
#9836=DIRECTION('center_axis',(0.,0.,-1.));
#9837=DIRECTION('ref_axis',(1.,0.,0.));
#9838=DIRECTION('center_axis',(0.,0.,1.));
#9839=DIRECTION('ref_axis',(1.,0.,0.));
#9840=DIRECTION('center_axis',(0.,0.,1.));
#9841=DIRECTION('ref_axis',(1.,0.,0.));
#9842=DIRECTION('center_axis',(0.,0.,1.));
#9843=DIRECTION('ref_axis',(1.,0.,0.));
#9844=DIRECTION('',(0.,0.,1.));
#9845=DIRECTION('center_axis',(0.,0.,-1.));
#9846=DIRECTION('ref_axis',(1.,0.,0.));
#9847=DIRECTION('center_axis',(0.,0.,1.));
#9848=DIRECTION('ref_axis',(1.,0.,0.));
#9849=DIRECTION('center_axis',(0.,0.,1.));
#9850=DIRECTION('ref_axis',(1.,0.,0.));
#9851=DIRECTION('center_axis',(0.,0.,1.));
#9852=DIRECTION('ref_axis',(1.,0.,0.));
#9853=DIRECTION('',(0.,0.,1.));
#9854=DIRECTION('center_axis',(0.,0.,-1.));
#9855=DIRECTION('ref_axis',(1.,0.,0.));
#9856=DIRECTION('center_axis',(0.,0.,1.));
#9857=DIRECTION('ref_axis',(1.,0.,0.));
#9858=DIRECTION('center_axis',(0.,0.,1.));
#9859=DIRECTION('ref_axis',(1.,0.,0.));
#9860=DIRECTION('',(0.,0.,-1.));
#9861=DIRECTION('center_axis',(0.,0.,1.));
#9862=DIRECTION('ref_axis',(1.,0.,0.));
#9863=DIRECTION('',(0.,0.,1.));
#9864=DIRECTION('center_axis',(0.,0.,1.));
#9865=DIRECTION('ref_axis',(1.,0.,0.));
#9866=DIRECTION('center_axis',(0.,0.,1.));
#9867=DIRECTION('ref_axis',(1.,0.,0.));
#9868=DIRECTION('center_axis',(0.,0.,1.));
#9869=DIRECTION('ref_axis',(1.,0.,0.));
#9870=DIRECTION('center_axis',(0.,0.,1.));
#9871=DIRECTION('ref_axis',(1.,0.,0.));
#9872=DIRECTION('',(0.,0.,-1.));
#9873=DIRECTION('center_axis',(0.,0.,1.));
#9874=DIRECTION('ref_axis',(1.,0.,0.));
#9875=DIRECTION('',(0.,0.,1.));
#9876=DIRECTION('center_axis',(0.,0.,1.));
#9877=DIRECTION('ref_axis',(1.,0.,0.));
#9878=DIRECTION('center_axis',(0.,0.,1.));
#9879=DIRECTION('ref_axis',(1.,0.,0.));
#9880=DIRECTION('center_axis',(0.,0.,1.));
#9881=DIRECTION('ref_axis',(1.,0.,0.));
#9882=DIRECTION('center_axis',(0.,0.,1.));
#9883=DIRECTION('ref_axis',(-0.707106781186548,-0.707106781186547,0.));
#9884=DIRECTION('',(0.,0.,-1.));
#9885=DIRECTION('center_axis',(0.,0.,1.));
#9886=DIRECTION('ref_axis',(1.,0.,0.));
#9887=DIRECTION('',(0.,0.,1.));
#9888=DIRECTION('center_axis',(0.,0.,1.));
#9889=DIRECTION('ref_axis',(1.,0.,0.));
#9890=DIRECTION('center_axis',(0.,0.,1.));
#9891=DIRECTION('ref_axis',(1.,0.,0.));
#9892=DIRECTION('center_axis',(0.,0.,1.));
#9893=DIRECTION('ref_axis',(1.,0.,0.));
#9894=DIRECTION('center_axis',(0.,0.,1.));
#9895=DIRECTION('ref_axis',(-0.707106781186547,0.707106781186548,0.));
#9896=DIRECTION('',(0.,0.,-1.));
#9897=DIRECTION('center_axis',(0.,0.,1.));
#9898=DIRECTION('ref_axis',(1.,0.,0.));
#9899=DIRECTION('',(0.,0.,1.));
#9900=DIRECTION('center_axis',(0.,0.,1.));
#9901=DIRECTION('ref_axis',(1.,0.,0.));
#9902=DIRECTION('center_axis',(0.,0.,1.));
#9903=DIRECTION('ref_axis',(1.,0.,0.));
#9904=DIRECTION('center_axis',(0.,0.,1.));
#9905=DIRECTION('ref_axis',(1.,0.,0.));
#9906=DIRECTION('center_axis',(0.,0.,1.));
#9907=DIRECTION('ref_axis',(1.,0.,0.));
#9908=DIRECTION('center_axis',(0.,0.,1.));
#9909=DIRECTION('ref_axis',(1.,0.,0.));
#9910=DIRECTION('center_axis',(0.,0.,1.));
#9911=DIRECTION('ref_axis',(1.,0.,0.));
#9912=DIRECTION('center_axis',(0.,0.,1.));
#9913=DIRECTION('ref_axis',(1.,0.,0.));
#9914=DIRECTION('center_axis',(0.,0.,1.));
#9915=DIRECTION('ref_axis',(1.,0.,0.));
#9916=DIRECTION('center_axis',(0.,0.,1.));
#9917=DIRECTION('ref_axis',(1.,0.,0.));
#9918=DIRECTION('center_axis',(0.,0.,1.));
#9919=DIRECTION('ref_axis',(1.,0.,0.));
#9920=DIRECTION('center_axis',(0.,0.,-1.));
#9921=DIRECTION('ref_axis',(1.,0.,0.));
#9922=DIRECTION('center_axis',(0.,0.,-1.));
#9923=DIRECTION('ref_axis',(1.,0.,0.));
#9924=DIRECTION('center_axis',(0.,0.,-1.));
#9925=DIRECTION('ref_axis',(1.,0.,0.));
#9926=DIRECTION('center_axis',(0.,0.,-1.));
#9927=DIRECTION('ref_axis',(1.,0.,0.));
#9928=DIRECTION('center_axis',(0.,0.,1.));
#9929=DIRECTION('ref_axis',(1.,0.,0.));
#9930=DIRECTION('center_axis',(0.,0.,1.));
#9931=DIRECTION('ref_axis',(1.,0.,0.));
#9932=DIRECTION('',(0.,0.,1.));
#9933=DIRECTION('center_axis',(0.,0.,1.));
#9934=DIRECTION('ref_axis',(1.,0.,0.));
#9935=DIRECTION('center_axis',(0.,0.,1.));
#9936=DIRECTION('ref_axis',(1.,0.,0.));
#9937=DIRECTION('',(0.,0.,1.));
#9938=DIRECTION('center_axis',(0.,0.,1.));
#9939=DIRECTION('ref_axis',(1.,0.,0.));
#9940=DIRECTION('center_axis',(0.,0.,1.));
#9941=DIRECTION('ref_axis',(1.,0.,0.));
#9942=DIRECTION('',(0.,0.,1.));
#9943=DIRECTION('center_axis',(0.,0.,1.));
#9944=DIRECTION('ref_axis',(1.,0.,0.));
#9945=DIRECTION('center_axis',(0.,0.,1.));
#9946=DIRECTION('ref_axis',(1.,0.,0.));
#9947=DIRECTION('',(0.,0.,1.));
#9948=DIRECTION('center_axis',(0.,0.,1.));
#9949=DIRECTION('ref_axis',(1.,0.,0.));
#9950=DIRECTION('center_axis',(0.,0.,1.));
#9951=DIRECTION('ref_axis',(1.,0.,0.));
#9952=DIRECTION('',(0.,0.,-1.));
#9953=DIRECTION('center_axis',(0.,0.,1.));
#9954=DIRECTION('ref_axis',(1.,0.,0.));
#9955=DIRECTION('center_axis',(0.,0.,1.));
#9956=DIRECTION('ref_axis',(1.,0.,0.));
#9957=DIRECTION('',(0.,0.,1.));
#9958=DIRECTION('center_axis',(0.,0.,-1.));
#9959=DIRECTION('ref_axis',(1.,0.,0.));
#9960=DIRECTION('center_axis',(0.,0.,1.));
#9961=DIRECTION('ref_axis',(1.,0.,0.));
#9962=DIRECTION('center_axis',(0.,0.,1.));
#9963=DIRECTION('ref_axis',(1.,0.,0.));
#9964=DIRECTION('center_axis',(0.,0.,1.));
#9965=DIRECTION('ref_axis',(1.,0.,0.));
#9966=DIRECTION('',(0.,0.,-1.));
#9967=DIRECTION('center_axis',(0.,0.,1.));
#9968=DIRECTION('ref_axis',(1.,0.,0.));
#9969=DIRECTION('center_axis',(0.,0.,1.));
#9970=DIRECTION('ref_axis',(1.,0.,0.));
#9971=DIRECTION('',(0.,0.,-1.));
#9972=DIRECTION('center_axis',(0.,0.,-1.));
#9973=DIRECTION('ref_axis',(1.,0.,0.));
#9974=DIRECTION('center_axis',(0.,0.,1.));
#9975=DIRECTION('ref_axis',(1.,0.,0.));
#9976=DIRECTION('center_axis',(0.,0.,1.));
#9977=DIRECTION('ref_axis',(1.,0.,0.));
#12382=CARTESIAN_POINT('',(0.,0.,0.));
#12383=CARTESIAN_POINT('Origin',(0.9,6.,1.4));
#12384=CARTESIAN_POINT('',(0.988888264668967,6.25,1.4));
#12385=CARTESIAN_POINT('',(1.02,6.,1.65));
#12386=CARTESIAN_POINT('Ctrl Pts',(0.988888264668967,6.25,1.4));
#12387=CARTESIAN_POINT('Ctrl Pts',(0.988888264668967,6.25,1.43153139415882));
#12388=CARTESIAN_POINT('Ctrl Pts',(0.990553370646674,6.2436720484314,1.46507214966317));
#12389=CARTESIAN_POINT('Ctrl Pts',(0.996491737296663,6.21811983001438,1.52662620974954));
#12390=CARTESIAN_POINT('Ctrl Pts',(1.00067109353237,6.19890212820607,1.5546512623872));
#12391=CARTESIAN_POINT('Ctrl Pts',(1.00845756932386,6.15465411356872,1.59889927702456));
#12392=CARTESIAN_POINT('Ctrl Pts',(1.01258144235289,6.12662787094525,1.61811920309393));
#12393=CARTESIAN_POINT('Ctrl Pts',(1.0183917429657,6.06506960039136,1.64367304400768));
#12394=CARTESIAN_POINT('Ctrl Pts',(1.02,6.03152733088338,1.65));
#12395=CARTESIAN_POINT('Ctrl Pts',(1.02,6.,1.65));
#12396=CARTESIAN_POINT('Ctrl Pts',(1.02,6.,1.65));
#12397=CARTESIAN_POINT('Ctrl Pts',(1.02,5.96847266911662,1.65));
#12398=CARTESIAN_POINT('Ctrl Pts',(1.0183917429657,5.93493039960864,1.64367304400768));
#12399=CARTESIAN_POINT('Ctrl Pts',(1.01258144235289,5.87337212905475,1.61811920309393));
#12400=CARTESIAN_POINT('Ctrl Pts',(1.00845756932386,5.84534588643128,1.59889927702456));
#12401=CARTESIAN_POINT('Ctrl Pts',(1.00067109353237,5.80109787179393,1.5546512623872));
#12402=CARTESIAN_POINT('Ctrl Pts',(0.996491737296663,5.78188016998562,1.52662620974954));
#12403=CARTESIAN_POINT('Ctrl Pts',(0.990553370646674,5.7563279515686,1.46507214966317));
#12404=CARTESIAN_POINT('Ctrl Pts',(0.988888264668967,5.75,1.43153139415882));
#12405=CARTESIAN_POINT('Ctrl Pts',(0.988888264668967,5.75,1.36846860584118));
#12406=CARTESIAN_POINT('Ctrl Pts',(0.990553370646674,5.7563279515686,1.33492785033683));
#12407=CARTESIAN_POINT('Ctrl Pts',(0.996491737296663,5.78188016998562,1.27337379025046));
#12408=CARTESIAN_POINT('Ctrl Pts',(1.00067109353237,5.80109787179393,1.2453487376128));
#12409=CARTESIAN_POINT('Ctrl Pts',(1.00845756932386,5.84534588643128,1.20110072297544));
#12410=CARTESIAN_POINT('Ctrl Pts',(1.01258144235289,5.87337212905475,1.18188079690607));
#12411=CARTESIAN_POINT('Ctrl Pts',(1.0183917429657,5.93493039960864,1.15632695599232));
#12412=CARTESIAN_POINT('Ctrl Pts',(1.02,5.96847266911662,1.15));
#12413=CARTESIAN_POINT('Ctrl Pts',(1.02,6.03152733088338,1.15));
#12414=CARTESIAN_POINT('Ctrl Pts',(1.0183917429657,6.06506960039136,1.15632695599232));
#12415=CARTESIAN_POINT('Ctrl Pts',(1.01258144235289,6.12662787094525,1.18188079690607));
#12416=CARTESIAN_POINT('Ctrl Pts',(1.00845756932386,6.15465411356872,1.20110072297544));
#12417=CARTESIAN_POINT('Ctrl Pts',(1.00067109353237,6.19890212820607,1.2453487376128));
#12418=CARTESIAN_POINT('Ctrl Pts',(0.996491737296663,6.21811983001438,1.27337379025046));
#12419=CARTESIAN_POINT('Ctrl Pts',(0.990553370646674,6.2436720484314,1.33492785033683));
#12420=CARTESIAN_POINT('Ctrl Pts',(0.988888264668967,6.25,1.36846860584118));
#12421=CARTESIAN_POINT('Ctrl Pts',(0.988888264668967,6.25,1.4));
#12422=CARTESIAN_POINT('',(2.9,6.,1.65));
#12423=CARTESIAN_POINT('',(0.9,6.,1.65));
#12424=CARTESIAN_POINT('',(2.88920404263873,6.25,1.4));
#12425=CARTESIAN_POINT('Ctrl Pts',(2.88920404263873,6.25,1.4));
#12426=CARTESIAN_POINT('Ctrl Pts',(2.88920404263873,6.25,1.36859268214333));
#12427=CARTESIAN_POINT('Ctrl Pts',(2.8897689135262,6.24372004673696,1.33510260402868));
#12428=CARTESIAN_POINT('Ctrl Pts',(2.89180770664292,6.21820179201259,1.27351240469396));
#12429=CARTESIAN_POINT('Ctrl Pts',(2.89325203146722,6.19896434419768,1.24541095360441));
#12430=CARTESIAN_POINT('Ctrl Pts',(2.89596207500507,6.15458908800492,1.20103569741165));
#12431=CARTESIAN_POINT('Ctrl Pts',(2.89740405468483,6.12648761856264,1.18179821727708));
#12432=CARTESIAN_POINT('Ctrl Pts',(2.89943748106926,6.06489735826727,1.15627993798745));
#12433=CARTESIAN_POINT('Ctrl Pts',(2.9,6.03140725895734,1.15));
#12434=CARTESIAN_POINT('Ctrl Pts',(2.9,5.96859274104266,1.15));
#12435=CARTESIAN_POINT('Ctrl Pts',(2.89943748106926,5.93510264173273,1.15627993798745));
#12436=CARTESIAN_POINT('Ctrl Pts',(2.89740405468483,5.87351238143735,1.18179821727708));
#12437=CARTESIAN_POINT('Ctrl Pts',(2.89596207500507,5.84541091199508,1.20103569741165));
#12438=CARTESIAN_POINT('Ctrl Pts',(2.89325203146722,5.80103565580232,1.24541095360441));
#12439=CARTESIAN_POINT('Ctrl Pts',(2.89180770664292,5.78179820798741,1.27351240469396));
#12440=CARTESIAN_POINT('Ctrl Pts',(2.8897689135262,5.75627995326304,1.33510260402868));
#12441=CARTESIAN_POINT('Ctrl Pts',(2.88920404263873,5.75,1.36859268214333));
#12442=CARTESIAN_POINT('Ctrl Pts',(2.88920404263873,5.75,1.43140731785667));
#12443=CARTESIAN_POINT('Ctrl Pts',(2.8897689135262,5.75627995326304,1.46489739597132));
#12444=CARTESIAN_POINT('Ctrl Pts',(2.89180770664292,5.78179820798741,1.52648759530604));
#12445=CARTESIAN_POINT('Ctrl Pts',(2.89325203146722,5.80103565580232,1.55458904639559));
#12446=CARTESIAN_POINT('Ctrl Pts',(2.89596207500507,5.84541091199508,1.59896430258835));
#12447=CARTESIAN_POINT('Ctrl Pts',(2.89740405468483,5.87351238143735,1.61820178272292));
#12448=CARTESIAN_POINT('Ctrl Pts',(2.89943748106926,5.93510264173273,1.64372006201255));
#12449=CARTESIAN_POINT('Ctrl Pts',(2.9,5.96859274104266,1.65));
#12450=CARTESIAN_POINT('Ctrl Pts',(2.9,6.,1.65));
#12451=CARTESIAN_POINT('Ctrl Pts',(2.9,6.,1.65));
#12452=CARTESIAN_POINT('Ctrl Pts',(2.9,6.03140725895734,1.65));
#12453=CARTESIAN_POINT('Ctrl Pts',(2.89943748106926,6.06489735826727,1.64372006201255));
#12454=CARTESIAN_POINT('Ctrl Pts',(2.89740405468483,6.12648761856265,1.61820178272292));
#12455=CARTESIAN_POINT('Ctrl Pts',(2.89596207500507,6.15458908800492,1.59896430258835));
#12456=CARTESIAN_POINT('Ctrl Pts',(2.89325203146722,6.19896434419768,1.55458904639559));
#12457=CARTESIAN_POINT('Ctrl Pts',(2.89180770664292,6.21820179201259,1.52648759530604));
#12458=CARTESIAN_POINT('Ctrl Pts',(2.8897689135262,6.24372004673696,1.46489739597132));
#12459=CARTESIAN_POINT('Ctrl Pts',(2.88920404263873,6.25,1.43140731785667));
#12460=CARTESIAN_POINT('Ctrl Pts',(2.88920404263873,6.25,1.4));
#12461=CARTESIAN_POINT('Origin',(-1.23743686707646,4.76256313292354,2.9));
#12462=CARTESIAN_POINT('',(-1.40243686707646,4.76256313292354,2.9));
#12463=CARTESIAN_POINT('Origin',(-1.23743686707646,4.76256313292354,2.9));
#12464=CARTESIAN_POINT('',(-1.40243686707646,4.76256313292354,3.6));
#12465=CARTESIAN_POINT('',(-1.40243686707646,4.76256313292354,2.9));
#12466=CARTESIAN_POINT('Origin',(-1.23743686707646,4.76256313292354,3.6));
#12467=CARTESIAN_POINT('Origin',(-1.23743686707646,4.76256313292354,2.9));
#12468=CARTESIAN_POINT('Origin',(-1.23743686707646,7.23743686707646,2.9));
#12469=CARTESIAN_POINT('',(-1.40243686707646,7.23743686707646,2.9));
#12470=CARTESIAN_POINT('Origin',(-1.23743686707646,7.23743686707646,2.9));
#12471=CARTESIAN_POINT('',(-1.40243686707646,7.23743686707646,3.6));
#12472=CARTESIAN_POINT('',(-1.40243686707646,7.23743686707646,2.9));
#12473=CARTESIAN_POINT('Origin',(-1.23743686707646,7.23743686707646,3.6));
#12474=CARTESIAN_POINT('Origin',(-1.23743686707646,7.23743686707646,2.9));
#12475=CARTESIAN_POINT('Origin',(1.23743686707646,7.23743686707646,2.9));
#12476=CARTESIAN_POINT('',(1.07243686707646,7.23743686707646,2.9));
#12477=CARTESIAN_POINT('Origin',(1.23743686707646,7.23743686707646,2.9));
#12478=CARTESIAN_POINT('',(1.07243686707646,7.23743686707646,3.6));
#12479=CARTESIAN_POINT('',(1.07243686707646,7.23743686707646,2.9));
#12480=CARTESIAN_POINT('Origin',(1.23743686707646,7.23743686707646,3.6));
#12481=CARTESIAN_POINT('Origin',(1.23743686707646,7.23743686707646,2.9));
#12482=CARTESIAN_POINT('Origin',(1.23743686707646,4.76256313292354,2.9));
#12483=CARTESIAN_POINT('',(1.07243686707646,4.76256313292354,2.9));
#12484=CARTESIAN_POINT('Origin',(1.23743686707646,4.76256313292354,2.9));
#12485=CARTESIAN_POINT('',(1.07243686707646,4.76256313292354,3.6));
#12486=CARTESIAN_POINT('',(1.07243686707646,4.76256313292354,2.9));
#12487=CARTESIAN_POINT('Origin',(1.23743686707646,4.76256313292354,3.6));
#12488=CARTESIAN_POINT('Origin',(1.23743686707646,4.76256313292354,2.9));
#12489=CARTESIAN_POINT('Origin',(-1.69705627484771,4.30294372515229,1.8));
#12490=CARTESIAN_POINT('',(-1.19413676298012,4.15228860714143,2.4));
#12491=CARTESIAN_POINT('',(-1.19413676298012,4.15228860714143,1.8));
#12492=CARTESIAN_POINT('',(-1.19413676298012,4.15228860714143,1.8));
#12493=CARTESIAN_POINT('',(-1.84771139285857,4.80586323701988,2.4));
#12494=CARTESIAN_POINT('Origin',(-1.69705627484771,4.30294372515229,2.4));
#12495=CARTESIAN_POINT('',(-1.84771139285857,4.80586323701988,1.8));
#12496=CARTESIAN_POINT('',(-1.84771139285857,4.80586323701988,1.8));
#12497=CARTESIAN_POINT('Origin',(-1.69705627484771,4.30294372515229,1.8));
#12498=CARTESIAN_POINT('Origin',(-1.69705627484771,4.30294372515229,2.4));
#12499=CARTESIAN_POINT('Origin',(0.,6.,2.4));
#12500=CARTESIAN_POINT('Origin',(-1.69705627484771,7.69705627484771,1.8));
#12501=CARTESIAN_POINT('',(-1.84771139285857,7.19413676298012,2.4));
#12502=CARTESIAN_POINT('',(-1.84771139285857,7.19413676298012,1.8));
#12503=CARTESIAN_POINT('',(-1.84771139285857,7.19413676298012,1.8));
#12504=CARTESIAN_POINT('',(-1.19413676298012,7.84771139285857,2.4));
#12505=CARTESIAN_POINT('Origin',(-1.69705627484771,7.69705627484771,2.4));
#12506=CARTESIAN_POINT('',(-1.19413676298012,7.84771139285857,1.8));
#12507=CARTESIAN_POINT('',(-1.19413676298012,7.84771139285857,1.8));
#12508=CARTESIAN_POINT('Origin',(-1.69705627484771,7.69705627484771,1.8));
#12509=CARTESIAN_POINT('Origin',(-1.69705627484771,7.69705627484771,2.4));
#12510=CARTESIAN_POINT('Origin',(0.,6.,2.4));
#12511=CARTESIAN_POINT('Origin',(1.69705627484771,7.69705627484771,1.8));
#12512=CARTESIAN_POINT('',(1.19413676298012,7.84771139285857,2.4));
#12513=CARTESIAN_POINT('',(1.19413676298012,7.84771139285857,1.8));
#12514=CARTESIAN_POINT('',(1.19413676298012,7.84771139285857,1.8));
#12515=CARTESIAN_POINT('',(1.84771139285857,7.19413676298012,2.4));
#12516=CARTESIAN_POINT('Origin',(1.69705627484771,7.69705627484771,2.4));
#12517=CARTESIAN_POINT('',(1.84771139285857,7.19413676298012,1.8));
#12518=CARTESIAN_POINT('',(1.84771139285857,7.19413676298012,1.8));
#12519=CARTESIAN_POINT('Origin',(1.69705627484771,7.69705627484771,1.8));
#12520=CARTESIAN_POINT('Origin',(1.69705627484771,7.69705627484771,2.4));
#12521=CARTESIAN_POINT('Origin',(0.,6.,2.4));
#12522=CARTESIAN_POINT('Origin',(1.69705627484771,4.30294372515229,1.8));
#12523=CARTESIAN_POINT('',(1.84771139285857,4.80586323701988,2.4));
#12524=CARTESIAN_POINT('',(1.84771139285857,4.80586323701988,1.8));
#12525=CARTESIAN_POINT('',(1.84771139285857,4.80586323701988,1.8));
#12526=CARTESIAN_POINT('',(1.19413676298012,4.15228860714143,2.4));
#12527=CARTESIAN_POINT('Origin',(1.69705627484771,4.30294372515229,2.4));
#12528=CARTESIAN_POINT('',(1.19413676298012,4.15228860714143,1.8));
#12529=CARTESIAN_POINT('',(1.19413676298012,4.15228860714143,1.8));
#12530=CARTESIAN_POINT('Origin',(1.69705627484771,4.30294372515229,1.8));
#12531=CARTESIAN_POINT('Origin',(1.69705627484771,4.30294372515229,2.4));
#12532=CARTESIAN_POINT('Origin',(0.,6.,2.4));
#12533=CARTESIAN_POINT('Origin',(0.,6.,1.8));
#12534=CARTESIAN_POINT('',(-2.9,6.,1.8));
#12535=CARTESIAN_POINT('Origin',(0.,6.,1.8));
#12536=CARTESIAN_POINT('',(-2.2,6.,1.8));
#12537=CARTESIAN_POINT('Origin',(0.,6.,1.8));
#12538=CARTESIAN_POINT('Origin',(0.,6.,1.8));
#12539=CARTESIAN_POINT('Origin',(0.,6.,1.8));
#12540=CARTESIAN_POINT('Origin',(0.,6.,1.8));
#12541=CARTESIAN_POINT('Origin',(0.,6.,1.8));
#12542=CARTESIAN_POINT('',(-1.97205627484771,4.30294372515229,1.8));
#12543=CARTESIAN_POINT('Origin',(-1.69705627484771,4.30294372515229,1.8));
#12544=CARTESIAN_POINT('',(-1.97205627484771,7.69705627484771,1.8));
#12545=CARTESIAN_POINT('Origin',(-1.69705627484771,7.69705627484771,1.8));
#12546=CARTESIAN_POINT('',(1.42205627484771,7.69705627484771,1.8));
#12547=CARTESIAN_POINT('Origin',(1.69705627484771,7.69705627484771,1.8));
#12548=CARTESIAN_POINT('',(1.42205627484771,4.30294372515229,1.8));
#12549=CARTESIAN_POINT('Origin',(1.69705627484771,4.30294372515229,1.8));
#12550=CARTESIAN_POINT('Origin',(-1.69705627484771,4.30294372515229,0.9));
#12551=CARTESIAN_POINT('',(-1.97205627484771,4.30294372515229,1.));
#12552=CARTESIAN_POINT('Origin',(-1.69705627484771,4.30294372515229,1.));
#12553=CARTESIAN_POINT('',(-1.97205627484771,4.30294372515229,0.9));
#12554=CARTESIAN_POINT('Origin',(-1.69705627484771,7.69705627484771,0.9));
#12555=CARTESIAN_POINT('',(-1.97205627484771,7.69705627484771,1.));
#12556=CARTESIAN_POINT('Origin',(-1.69705627484771,7.69705627484771,1.));
#12557=CARTESIAN_POINT('',(-1.97205627484771,7.69705627484771,0.9));
#12558=CARTESIAN_POINT('Origin',(1.69705627484771,7.69705627484771,0.9));
#12559=CARTESIAN_POINT('',(1.42205627484771,7.69705627484771,1.));
#12560=CARTESIAN_POINT('Origin',(1.69705627484771,7.69705627484771,1.));
#12561=CARTESIAN_POINT('',(1.42205627484771,7.69705627484771,0.9));
#12562=CARTESIAN_POINT('Origin',(1.69705627484771,4.30294372515229,0.9));
#12563=CARTESIAN_POINT('',(1.42205627484771,4.30294372515229,1.));
#12564=CARTESIAN_POINT('Origin',(1.69705627484771,4.30294372515229,1.));
#12565=CARTESIAN_POINT('',(1.42205627484771,4.30294372515229,0.9));
#12566=CARTESIAN_POINT('Origin',(0.,6.,1.));
#12567=CARTESIAN_POINT('',(-2.2,6.,3.6));
#12568=CARTESIAN_POINT('Origin',(0.,6.,3.6));
#12569=CARTESIAN_POINT('',(-2.2,6.,1.));
#12570=CARTESIAN_POINT('Origin',(0.,6.,2.05));
#12571=CARTESIAN_POINT('',(-1.5,6.,2.05));
#12572=CARTESIAN_POINT('Origin',(0.,6.,2.05));
#12573=CARTESIAN_POINT('',(-1.5,6.,3.6));
#12574=CARTESIAN_POINT('',(-1.5,6.,2.05));
#12575=CARTESIAN_POINT('Origin',(0.,6.,3.6));
#12576=CARTESIAN_POINT('Origin',(0.,6.,2.05));
#12577=CARTESIAN_POINT('',(-1.02,6.,2.05));
#12578=CARTESIAN_POINT('Origin',(0.,6.,2.05));
#12579=CARTESIAN_POINT('Origin',(0.,6.,1.));
#12580=CARTESIAN_POINT('',(-2.9,6.,1.));
#12581=CARTESIAN_POINT('',(-2.9,6.,1.));
#12582=CARTESIAN_POINT('Origin',(0.,6.,1.));
#12583=CARTESIAN_POINT('Origin',(0.,6.,1.));
#12584=CARTESIAN_POINT('',(-1.02,6.,1.));
#12585=CARTESIAN_POINT('',(-1.02,6.,1.));
#12586=CARTESIAN_POINT('Origin',(0.,6.,1.));
#12587=CARTESIAN_POINT('Origin',(0.,6.,3.6));
#12588=CARTESIAN_POINT('Origin',(0.,6.,1.));
#14778=UNCERTAINTY_MEASURE_WITH_UNIT(LENGTH_MEASURE(0.001),#14879,
'DISTANCE_ACCURACY_VALUE',
'Maximum model space distance between geometric entities at asserted c
onnectivities');
#14824=UNCERTAINTY_MEASURE_WITH_UNIT(LENGTH_MEASURE(0.001),#14879,
'DISTANCE_ACCURACY_VALUE',
'Maximum model space distance between geometric entities at asserted c
onnectivities');
#14832=(
GEOMETRIC_REPRESENTATION_CONTEXT(3)
GLOBAL_UNCERTAINTY_ASSIGNED_CONTEXT((#14778))
GLOBAL_UNIT_ASSIGNED_CONTEXT((#14879,#14881,#14882))
REPRESENTATION_CONTEXT('','3D')
);
#14878=(
GEOMETRIC_REPRESENTATION_CONTEXT(3)
GLOBAL_UNCERTAINTY_ASSIGNED_CONTEXT((#14824))
GLOBAL_UNIT_ASSIGNED_CONTEXT((#14879,#14881,#14882))
REPRESENTATION_CONTEXT('','3D')
);
#14879=(
LENGTH_UNIT()
NAMED_UNIT(*)
SI_UNIT(.CENTI.,.METRE.)
);
#14881=(
NAMED_UNIT(*)
PLANE_ANGLE_UNIT()
SI_UNIT($,.RADIAN.)
);
#14882=(
NAMED_UNIT(*)
SI_UNIT($,.STERADIAN.)
SOLID_ANGLE_UNIT()
);
#14890=SHAPE_DEFINITION_REPRESENTATION(#14943,#15075);
#14943=PRODUCT_DEFINITION_SHAPE('',$,#15129);
#15075=SHAPE_REPRESENTATION('',(#8554),#14832);
#15121=PRODUCT_DEFINITION_CONTEXT('part definition',#15282,'design');
#15129=PRODUCT_DEFINITION('Crank bearing post','Crank bearing post',#15182,
#15121);
#15182=PRODUCT_DEFINITION_FORMATION('',$,#15291);
#15282=APPLICATION_CONTEXT(
'Core Data for Automotive Mechanical Design Process');
#15283=PRODUCT_CONTEXT('part definition',#15282,'mechanical');
#15291=PRODUCT('Crank bearing post','Crank bearing post',
'Crank bearing post',(#15283));
#15400=COLOUR_RGB('Grey',0.48,0.52,0.57);
#15401=FILL_AREA_STYLE_COLOUR('',#15400);
#15402=FILL_AREA_STYLE('',(#15401));
#15403=SURFACE_STYLE_FILL_AREA(#15402);
#15404=SURFACE_SIDE_STYLE('',(#15403));
#15405=SURFACE_STYLE_USAGE(.BOTH.,#15404);
#15406=PRESENTATION_STYLE_ASSIGNMENT((#15405));
ENDSEC;
END-ISO-10303-21;
